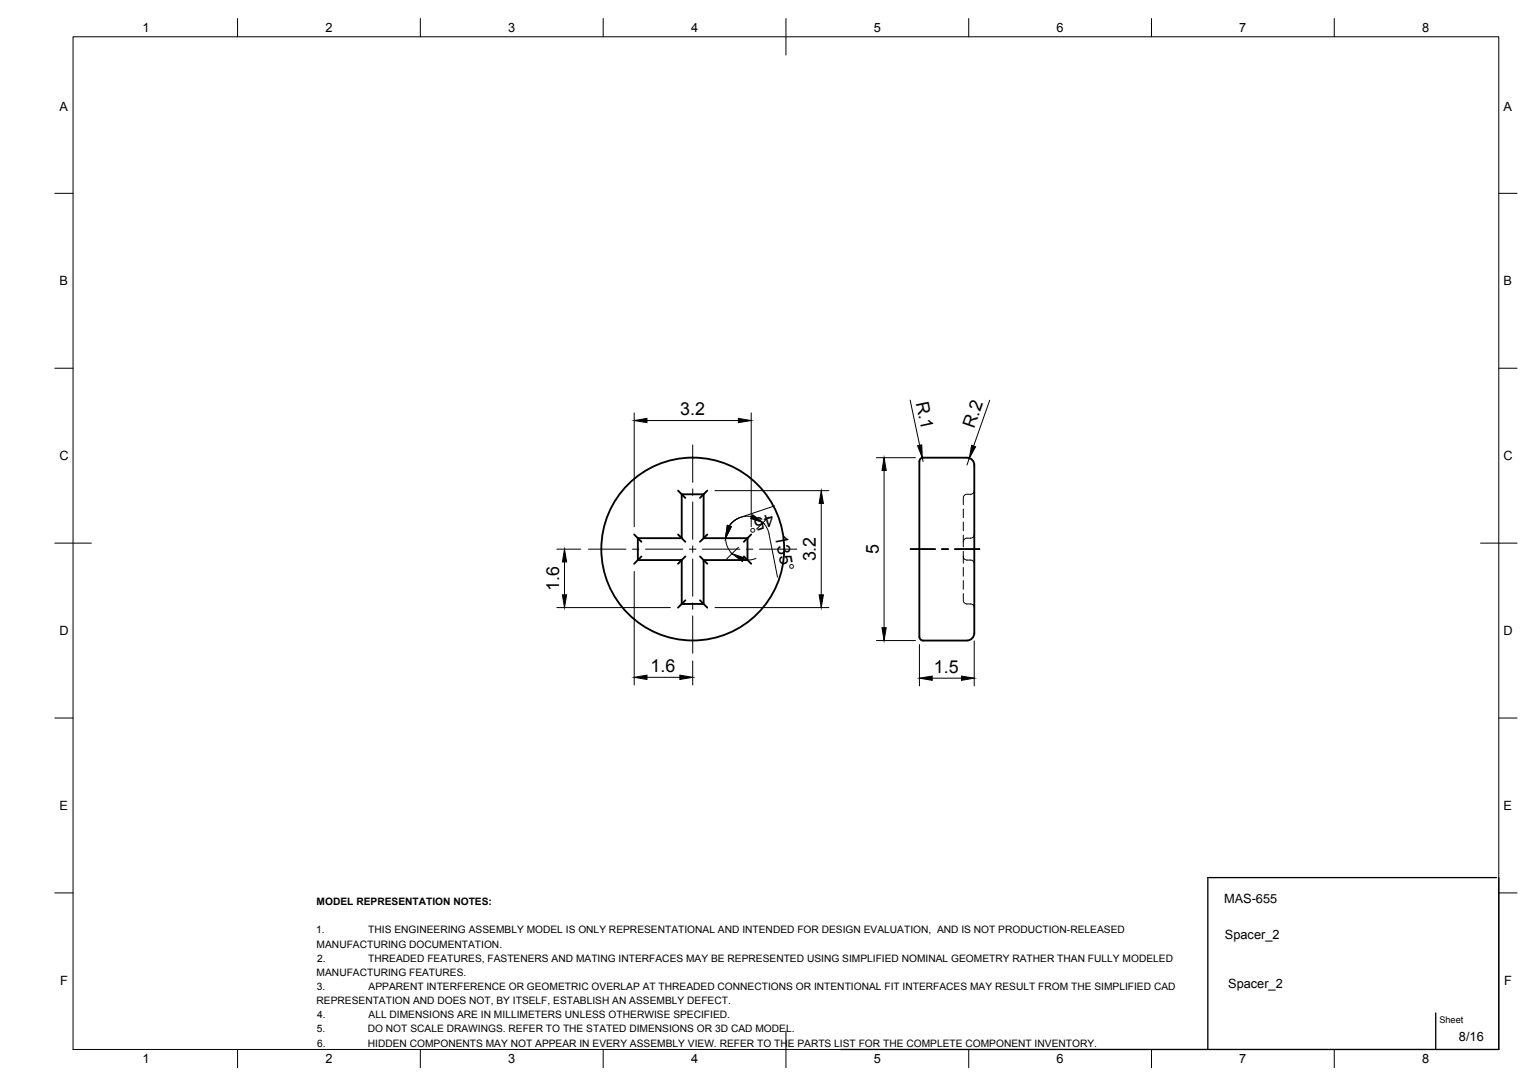
ISO-10303-21;
HEADER;
FILE_DESCRIPTION((''),'2;1');
FILE_NAME('Spacer_2.step','2026-10-09T11:34:15-07:00',(''),(''),'','','');
FILE_SCHEMA (('AUTOMOTIVE_DESIGN { 1 0 10303 214 3 1 1 }'));
ENDSEC;
DATA;
#10=MECHANICAL_DESIGN_GEOMETRIC_PRESENTATION_REPRESENTATION('',(#640),#117170);
#341=ELLIPSE('',#52296,0.141421356237297,0.1) ;
#342=ELLIPSE('',#52297,0.141421356237322,0.1) ;
#343=ELLIPSE('',#52299,0.141421356237322,0.1) ;
#344=ELLIPSE('',#52301,0.141421356237297,0.1) ;
#345=ELLIPSE('',#52303,0.141421356237322,0.1) ;
#346=ELLIPSE('',#52305,0.141421356237297,0.1) ;
#347=ELLIPSE('',#52307,0.141421356237322,0.1) ;
#348=ELLIPSE('',#52309,0.141421356237297,0.1) ;
#349=ELLIPSE('',#52311,0.141421356237322,0.1) ;
#350=ELLIPSE('',#52313,0.141421356237297,0.1) ;
#351=ELLIPSE('',#52315,0.141421356237322,0.1) ;
#352=ELLIPSE('',#52317,0.141421356237297,0.1) ;
#353=ELLIPSE('',#52336,0.141421356237297,0.1) ;
#354=ELLIPSE('',#52337,0.141421356237322,0.1) ;
#355=ELLIPSE('',#52339,0.141421356237322,0.1) ;
#356=ELLIPSE('',#52341,0.141421356237297,0.1) ;
#357=ELLIPSE('',#52343,0.141421356237322,0.1) ;
#358=ELLIPSE('',#52345,0.141421356237297,0.1) ;
#359=ELLIPSE('',#52347,0.141421356237297,0.1) ;
#360=ELLIPSE('',#52348,0.141421356237297,0.1) ;
#361=ELLIPSE('',#52350,0.141421356237322,0.1) ;
#362=ELLIPSE('',#52353,0.141421356237297,0.1) ;
#363=ELLIPSE('',#52355,0.141421356237322,0.1) ;
#364=ELLIPSE('',#52357,0.141421356237297,0.1) ;
#598=SHAPE_REPRESENTATION_RELATIONSHIP('SRR','None',#117253,#619) ;
#619=ADVANCED_BREP_SHAPE_REPRESENTATION('',(#661),#117161) ;
#640=STYLED_ITEM('',(#117355),#661) ;
#661=MANIFOLD_SOLID_BREP('Body1',#49069) ;
#735=FACE_BOUND('',#15452,.T.) ;
#2522=PLANE('',#52319) ;
#2523=PLANE('',#52320) ;
#2524=PLANE('',#52321) ;
#2525=PLANE('',#52322) ;
#2526=PLANE('',#52323) ;
#2527=PLANE('',#52324) ;
#2528=PLANE('',#52325) ;
#2529=PLANE('',#52334) ;
#2530=PLANE('',#52359) ;
#2531=PLANE('',#52360) ;
#2532=PLANE('',#52361) ;
#2533=PLANE('',#52362) ;
#2534=PLANE('',#52366) ;
#2535=PLANE('',#52367) ;
#2536=PLANE('',#52368) ;
#4427=LINE('',#88396,#7641) ;
#4428=LINE('',#88400,#7642) ;
#4429=LINE('',#88404,#7643) ;
#4430=LINE('',#88407,#7644) ;
#4431=LINE('',#88410,#7645) ;
#4432=LINE('',#88413,#7646) ;
#4433=LINE('',#88416,#7647) ;
#4434=LINE('',#88419,#7648) ;
#4435=LINE('',#88422,#7649) ;
#4436=LINE('',#88425,#7650) ;
#4437=LINE('',#88428,#7651) ;
#4438=LINE('',#88430,#7652) ;
#4439=LINE('',#88434,#7653) ;
#4440=LINE('',#88436,#7654) ;
#4441=LINE('',#88440,#7655) ;
#4442=LINE('',#88442,#7656) ;
#4443=LINE('',#88446,#7657) ;
#4444=LINE('',#88448,#7658) ;
#4445=LINE('',#88452,#7659) ;
#4446=LINE('',#88454,#7660) ;
#4447=LINE('',#88458,#7661) ;
#4448=LINE('',#88460,#7662) ;
#4449=LINE('',#88463,#7663) ;
#4450=LINE('',#88464,#7664) ;
#4451=LINE('',#88467,#7665) ;
#4452=LINE('',#88469,#7666) ;
#4453=LINE('',#88470,#7667) ;
#4454=LINE('',#88473,#7668) ;
#4455=LINE('',#88474,#7669) ;
#4456=LINE('',#88477,#7670) ;
#4457=LINE('',#88478,#7671) ;
#4458=LINE('',#88481,#7672) ;
#4459=LINE('',#88482,#7673) ;
#4460=LINE('',#88485,#7674) ;
#4461=LINE('',#88486,#7675) ;
#4462=LINE('',#88489,#7676) ;
#4463=LINE('',#88490,#7677) ;
#4464=LINE('',#88502,#7678) ;
#4465=LINE('',#88510,#7679) ;
#4466=LINE('',#88515,#7680) ;
#4467=LINE('',#88519,#7681) ;
#4468=LINE('',#88523,#7682) ;
#4469=LINE('',#88527,#7683) ;
#4470=LINE('',#88530,#7684) ;
#4471=LINE('',#88534,#7685) ;
#4472=LINE('',#88538,#7686) ;
#4473=LINE('',#88542,#7687) ;
#4474=LINE('',#88544,#7688) ;
#4475=LINE('',#88547,#7689) ;
#4476=LINE('',#88548,#7690) ;
#4477=LINE('',#88551,#7691) ;
#4478=LINE('',#88553,#7692) ;
#4479=LINE('',#88556,#7693) ;
#4480=LINE('',#88558,#7694) ;
#4481=LINE('',#88562,#7695) ;
#4482=LINE('',#88565,#7696) ;
#4483=LINE('',#88567,#7697) ;
#4484=LINE('',#88569,#7698) ;
#4485=LINE('',#88571,#7699) ;
#4486=LINE('',#88578,#7700) ;
#4487=LINE('',#88580,#7701) ;
#7641=VECTOR('',#62464,10.) ;
#7642=VECTOR('',#62467,10.) ;
#7643=VECTOR('',#62472,10.) ;
#7644=VECTOR('',#62475,10.) ;
#7645=VECTOR('',#62478,10.) ;
#7646=VECTOR('',#62481,10.) ;
#7647=VECTOR('',#62484,10.) ;
#7648=VECTOR('',#62487,10.) ;
#7649=VECTOR('',#62490,10.) ;
#7650=VECTOR('',#62493,10.) ;
#7651=VECTOR('',#62496,10.) ;
#7652=VECTOR('',#62497,10.) ;
#7653=VECTOR('',#62502,10.) ;
#7654=VECTOR('',#62503,10.) ;
#7655=VECTOR('',#62508,10.) ;
#7656=VECTOR('',#62509,10.) ;
#7657=VECTOR('',#62514,10.) ;
#7658=VECTOR('',#62515,10.) ;
#7659=VECTOR('',#62520,10.) ;
#7660=VECTOR('',#62521,10.) ;
#7661=VECTOR('',#62526,10.) ;
#7662=VECTOR('',#62527,10.) ;
#7663=VECTOR('',#62532,10.) ;
#7664=VECTOR('',#62533,10.) ;
#7665=VECTOR('',#62536,10.) ;
#7666=VECTOR('',#62537,10.) ;
#7667=VECTOR('',#62538,10.) ;
#7668=VECTOR('',#62541,10.) ;
#7669=VECTOR('',#62542,10.) ;
#7670=VECTOR('',#62545,10.) ;
#7671=VECTOR('',#62546,10.) ;
#7672=VECTOR('',#62549,10.) ;
#7673=VECTOR('',#62550,10.) ;
#7674=VECTOR('',#62553,10.) ;
#7675=VECTOR('',#62554,10.) ;
#7676=VECTOR('',#62557,10.) ;
#7677=VECTOR('',#62558,10.) ;
#7678=VECTOR('',#62573,2.49999999999999) ;
#7679=VECTOR('',#62582,10.) ;
#7680=VECTOR('',#62589,10.) ;
#7681=VECTOR('',#62594,10.) ;
#7682=VECTOR('',#62599,10.) ;
#7683=VECTOR('',#62604,10.) ;
#7684=VECTOR('',#62607,10.) ;
#7685=VECTOR('',#62610,10.) ;
#7686=VECTOR('',#62613,10.) ;
#7687=VECTOR('',#62618,10.) ;
#7688=VECTOR('',#62619,10.) ;
#7689=VECTOR('',#62624,10.) ;
#7690=VECTOR('',#62625,10.) ;
#7691=VECTOR('',#62628,10.) ;
#7692=VECTOR('',#62629,10.) ;
#7693=VECTOR('',#62634,10.) ;
#7694=VECTOR('',#62635,10.) ;
#7695=VECTOR('',#62640,10.) ;
#7696=VECTOR('',#62645,10.) ;
#7697=VECTOR('',#62648,10.) ;
#7698=VECTOR('',#62651,10.) ;
#7699=VECTOR('',#62654,10.) ;
#7700=VECTOR('',#62665,10.) ;
#7701=VECTOR('',#62668,10.) ;
#10065=CYLINDRICAL_SURFACE('',#52295,0.1) ;
#10066=CYLINDRICAL_SURFACE('',#52298,0.1) ;
#10067=CYLINDRICAL_SURFACE('',#52300,0.1) ;
#10068=CYLINDRICAL_SURFACE('',#52302,0.1) ;
#10069=CYLINDRICAL_SURFACE('',#52304,0.1) ;
#10070=CYLINDRICAL_SURFACE('',#52306,0.1) ;
#10071=CYLINDRICAL_SURFACE('',#52308,0.1) ;
#10072=CYLINDRICAL_SURFACE('',#52310,0.1) ;
#10073=CYLINDRICAL_SURFACE('',#52312,0.1) ;
#10074=CYLINDRICAL_SURFACE('',#52314,0.1) ;
#10075=CYLINDRICAL_SURFACE('',#52316,0.1) ;
#10076=CYLINDRICAL_SURFACE('',#52318,0.1) ;
#10077=CYLINDRICAL_SURFACE('',#52331,2.49999999999999) ;
#10078=CYLINDRICAL_SURFACE('',#52335,0.1) ;
#10079=CYLINDRICAL_SURFACE('',#52338,0.1) ;
#10080=CYLINDRICAL_SURFACE('',#52340,0.1) ;
#10081=CYLINDRICAL_SURFACE('',#52342,0.1) ;
#10082=CYLINDRICAL_SURFACE('',#52344,0.1) ;
#10083=CYLINDRICAL_SURFACE('',#52346,0.1) ;
#10084=CYLINDRICAL_SURFACE('',#52349,0.1) ;
#10085=CYLINDRICAL_SURFACE('',#52351,0.1) ;
#10086=CYLINDRICAL_SURFACE('',#52352,0.1) ;
#10087=CYLINDRICAL_SURFACE('',#52354,0.1) ;
#10088=CYLINDRICAL_SURFACE('',#52356,0.1) ;
#10089=CYLINDRICAL_SURFACE('',#52358,0.1) ;
#12257=FACE_OUTER_BOUND('',#15414,.T.) ;
#12258=FACE_OUTER_BOUND('',#15415,.T.) ;
#12259=FACE_OUTER_BOUND('',#15416,.T.) ;
#12260=FACE_OUTER_BOUND('',#15417,.T.) ;
#12261=FACE_OUTER_BOUND('',#15418,.T.) ;
#12262=FACE_OUTER_BOUND('',#15419,.T.) ;
#12263=FACE_OUTER_BOUND('',#15420,.T.) ;
#12264=FACE_OUTER_BOUND('',#15421,.T.) ;
#12265=FACE_OUTER_BOUND('',#15422,.T.) ;
#12266=FACE_OUTER_BOUND('',#15423,.T.) ;
#12267=FACE_OUTER_BOUND('',#15424,.T.) ;
#12268=FACE_OUTER_BOUND('',#15425,.T.) ;
#12269=FACE_OUTER_BOUND('',#15426,.T.) ;
#12270=FACE_OUTER_BOUND('',#15427,.T.) ;
#12271=FACE_OUTER_BOUND('',#15428,.T.) ;
#12272=FACE_OUTER_BOUND('',#15429,.T.) ;
#12273=FACE_OUTER_BOUND('',#15430,.T.) ;
#12274=FACE_OUTER_BOUND('',#15431,.T.) ;
#12275=FACE_OUTER_BOUND('',#15432,.T.) ;
#12276=FACE_OUTER_BOUND('',#15433,.T.) ;
#12277=FACE_OUTER_BOUND('',#15434,.T.) ;
#12278=FACE_OUTER_BOUND('',#15435,.T.) ;
#12279=FACE_OUTER_BOUND('',#15436,.T.) ;
#12280=FACE_OUTER_BOUND('',#15437,.T.) ;
#12281=FACE_OUTER_BOUND('',#15438,.T.) ;
#12282=FACE_OUTER_BOUND('',#15439,.T.) ;
#12283=FACE_OUTER_BOUND('',#15440,.T.) ;
#12284=FACE_OUTER_BOUND('',#15441,.T.) ;
#12285=FACE_OUTER_BOUND('',#15442,.T.) ;
#12286=FACE_OUTER_BOUND('',#15443,.T.) ;
#12287=FACE_OUTER_BOUND('',#15444,.T.) ;
#12288=FACE_OUTER_BOUND('',#15445,.T.) ;
#12289=FACE_OUTER_BOUND('',#15446,.T.) ;
#12290=FACE_OUTER_BOUND('',#15447,.T.) ;
#12291=FACE_OUTER_BOUND('',#15448,.T.) ;
#12292=FACE_OUTER_BOUND('',#15449,.T.) ;
#12293=FACE_OUTER_BOUND('',#15450,.T.) ;
#12294=FACE_OUTER_BOUND('',#15451,.T.) ;
#12295=FACE_OUTER_BOUND('',#15453,.T.) ;
#12296=FACE_OUTER_BOUND('',#15454,.T.) ;
#12297=FACE_OUTER_BOUND('',#15455,.T.) ;
#12298=FACE_OUTER_BOUND('',#15456,.T.) ;
#15414=EDGE_LOOP('',(#37928,#37929,#37930,#37931)) ;
#15415=EDGE_LOOP('',(#37932,#37933,#37934,#37935)) ;
#15416=EDGE_LOOP('',(#37936,#37937,#37938,#37939)) ;
#15417=EDGE_LOOP('',(#37940,#37941,#37942,#37943)) ;
#15418=EDGE_LOOP('',(#37944,#37945,#37946,#37947)) ;
#15419=EDGE_LOOP('',(#37948,#37949,#37950,#37951)) ;
#15420=EDGE_LOOP('',(#37952,#37953,#37954,#37955)) ;
#15421=EDGE_LOOP('',(#37956,#37957,#37958,#37959)) ;
#15422=EDGE_LOOP('',(#37960,#37961,#37962,#37963)) ;
#15423=EDGE_LOOP('',(#37964,#37965,#37966,#37967)) ;
#15424=EDGE_LOOP('',(#37968,#37969,#37970,#37971)) ;
#15425=EDGE_LOOP('',(#37972,#37973,#37974,#37975)) ;
#15426=EDGE_LOOP('',(#37976,#37977,#37978,#37979)) ;
#15427=EDGE_LOOP('',(#37980,#37981,#37982,#37983)) ;
#15428=EDGE_LOOP('',(#37984,#37985,#37986,#37987)) ;
#15429=EDGE_LOOP('',(#37988,#37989,#37990,#37991)) ;
#15430=EDGE_LOOP('',(#37992,#37993,#37994,#37995)) ;
#15431=EDGE_LOOP('',(#37996,#37997,#37998,#37999)) ;
#15432=EDGE_LOOP('',(#38000,#38001,#38002,#38003,#38004,#38005,#38006,#38007,
#38008,#38009,#38010,#38011)) ;
#15433=EDGE_LOOP('',(#38012,#38013,#38014,#38015,#38016)) ;
#15434=EDGE_LOOP('',(#38017,#38018,#38019,#38020,#38021,#38022)) ;
#15435=EDGE_LOOP('',(#38023)) ;
#15436=EDGE_LOOP('',(#38024,#38025,#38026,#38027)) ;
#15437=EDGE_LOOP('',(#38028,#38029,#38030,#38031)) ;
#15438=EDGE_LOOP('',(#38032,#38033,#38034,#38035)) ;
#15439=EDGE_LOOP('',(#38036,#38037,#38038,#38039)) ;
#15440=EDGE_LOOP('',(#38040,#38041,#38042,#38043)) ;
#15441=EDGE_LOOP('',(#38044,#38045,#38046,#38047)) ;
#15442=EDGE_LOOP('',(#38048,#38049,#38050,#38051)) ;
#15443=EDGE_LOOP('',(#38052,#38053,#38054,#38055)) ;
#15444=EDGE_LOOP('',(#38056,#38057,#38058,#38059)) ;
#15445=EDGE_LOOP('',(#38060,#38061,#38062,#38063)) ;
#15446=EDGE_LOOP('',(#38064,#38065,#38066,#38067)) ;
#15447=EDGE_LOOP('',(#38068,#38069,#38070,#38071)) ;
#15448=EDGE_LOOP('',(#38072,#38073,#38074,#38075)) ;
#15449=EDGE_LOOP('',(#38076,#38077,#38078,#38079)) ;
#15450=EDGE_LOOP('',(#38080,#38081,#38082,#38083)) ;
#15451=EDGE_LOOP('',(#38084)) ;
#15452=EDGE_LOOP('',(#38085,#38086,#38087,#38088,#38089,#38090,#38091,#38092,
#38093,#38094,#38095,#38096)) ;
#15453=EDGE_LOOP('',(#38097,#38098,#38099,#38100,#38101)) ;
#15454=EDGE_LOOP('',(#38102,#38103,#38104,#38105)) ;
#15455=EDGE_LOOP('',(#38106,#38107,#38108,#38109)) ;
#15456=EDGE_LOOP('',(#38110,#38111,#38112,#38113)) ;
#18493=CIRCLE('',#52327,2.39999999999999) ;
#18494=CIRCLE('',#52328,0.1) ;
#18495=CIRCLE('',#52329,2.49999999999999) ;
#18496=CIRCLE('',#52330,2.49999999999999) ;
#18497=CIRCLE('',#52332,2.49999999999999) ;
#18498=CIRCLE('',#52333,2.49999999999999) ;
#18499=CIRCLE('',#52363,2.29999999999999) ;
#18500=CIRCLE('',#52365,0.2) ;
#21561=VERTEX_POINT('',#88394) ;
#21562=VERTEX_POINT('',#88395) ;
#21563=VERTEX_POINT('',#88397) ;
#21564=VERTEX_POINT('',#88399) ;
#21565=VERTEX_POINT('',#88403) ;
#21566=VERTEX_POINT('',#88405) ;
#21567=VERTEX_POINT('',#88409) ;
#21568=VERTEX_POINT('',#88411) ;
#21569=VERTEX_POINT('',#88415) ;
#21570=VERTEX_POINT('',#88417) ;
#21571=VERTEX_POINT('',#88421) ;
#21572=VERTEX_POINT('',#88423) ;
#21573=VERTEX_POINT('',#88427) ;
#21574=VERTEX_POINT('',#88429) ;
#21575=VERTEX_POINT('',#88433) ;
#21576=VERTEX_POINT('',#88435) ;
#21577=VERTEX_POINT('',#88439) ;
#21578=VERTEX_POINT('',#88441) ;
#21579=VERTEX_POINT('',#88445) ;
#21580=VERTEX_POINT('',#88447) ;
#21581=VERTEX_POINT('',#88451) ;
#21582=VERTEX_POINT('',#88453) ;
#21583=VERTEX_POINT('',#88457) ;
#21584=VERTEX_POINT('',#88459) ;
#21585=VERTEX_POINT('',#88466) ;
#21586=VERTEX_POINT('',#88468) ;
#21587=VERTEX_POINT('',#88472) ;
#21588=VERTEX_POINT('',#88476) ;
#21589=VERTEX_POINT('',#88480) ;
#21590=VERTEX_POINT('',#88484) ;
#21591=VERTEX_POINT('',#88488) ;
#21592=VERTEX_POINT('',#88493) ;
#21593=VERTEX_POINT('',#88495) ;
#21594=VERTEX_POINT('',#88497) ;
#21595=VERTEX_POINT('',#88501) ;
#21596=VERTEX_POINT('',#88503) ;
#21597=VERTEX_POINT('',#88508) ;
#21598=VERTEX_POINT('',#88509) ;
#21599=VERTEX_POINT('',#88514) ;
#21600=VERTEX_POINT('',#88518) ;
#21601=VERTEX_POINT('',#88522) ;
#21602=VERTEX_POINT('',#88526) ;
#21603=VERTEX_POINT('',#88528) ;
#21604=VERTEX_POINT('',#88532) ;
#21605=VERTEX_POINT('',#88533) ;
#21606=VERTEX_POINT('',#88535) ;
#21607=VERTEX_POINT('',#88537) ;
#21608=VERTEX_POINT('',#88541) ;
#21609=VERTEX_POINT('',#88543) ;
#21610=VERTEX_POINT('',#88550) ;
#21611=VERTEX_POINT('',#88552) ;
#21612=VERTEX_POINT('',#88557) ;
#21613=VERTEX_POINT('',#88561) ;
#21614=VERTEX_POINT('',#88573) ;
#27242=EDGE_CURVE('',#21561,#21562,#4427,.T.) ;
#27243=EDGE_CURVE('',#21562,#21563,#341,.T.) ;
#27244=EDGE_CURVE('',#21563,#21564,#4428,.T.) ;
#27245=EDGE_CURVE('',#21561,#21564,#342,.T.) ;
#27246=EDGE_CURVE('',#21562,#21565,#4429,.T.) ;
#27247=EDGE_CURVE('',#21565,#21566,#343,.T.) ;
#27248=EDGE_CURVE('',#21566,#21563,#4430,.T.) ;
#27249=EDGE_CURVE('',#21565,#21567,#4431,.T.) ;
#27250=EDGE_CURVE('',#21567,#21568,#344,.T.) ;
#27251=EDGE_CURVE('',#21568,#21566,#4432,.T.) ;
#27252=EDGE_CURVE('',#21567,#21569,#4433,.T.) ;
#27253=EDGE_CURVE('',#21569,#21570,#345,.T.) ;
#27254=EDGE_CURVE('',#21570,#21568,#4434,.T.) ;
#27255=EDGE_CURVE('',#21569,#21571,#4435,.T.) ;
#27256=EDGE_CURVE('',#21571,#21572,#346,.T.) ;
#27257=EDGE_CURVE('',#21572,#21570,#4436,.T.) ;
#27258=EDGE_CURVE('',#21573,#21572,#4437,.T.) ;
#27259=EDGE_CURVE('',#21571,#21574,#4438,.T.) ;
#27260=EDGE_CURVE('',#21574,#21573,#347,.T.) ;
#27261=EDGE_CURVE('',#21575,#21573,#4439,.T.) ;
#27262=EDGE_CURVE('',#21574,#21576,#4440,.T.) ;
#27263=EDGE_CURVE('',#21576,#21575,#348,.T.) ;
#27264=EDGE_CURVE('',#21577,#21575,#4441,.T.) ;
#27265=EDGE_CURVE('',#21576,#21578,#4442,.T.) ;
#27266=EDGE_CURVE('',#21578,#21577,#349,.T.) ;
#27267=EDGE_CURVE('',#21579,#21577,#4443,.T.) ;
#27268=EDGE_CURVE('',#21578,#21580,#4444,.T.) ;
#27269=EDGE_CURVE('',#21580,#21579,#350,.T.) ;
#27270=EDGE_CURVE('',#21581,#21579,#4445,.T.) ;
#27271=EDGE_CURVE('',#21580,#21582,#4446,.T.) ;
#27272=EDGE_CURVE('',#21582,#21581,#351,.T.) ;
#27273=EDGE_CURVE('',#21583,#21581,#4447,.T.) ;
#27274=EDGE_CURVE('',#21582,#21584,#4448,.T.) ;
#27275=EDGE_CURVE('',#21584,#21583,#352,.T.) ;
#27276=EDGE_CURVE('',#21564,#21583,#4449,.T.) ;
#27277=EDGE_CURVE('',#21584,#21561,#4450,.T.) ;
#27278=EDGE_CURVE('',#21585,#21577,#4451,.T.) ;
#27279=EDGE_CURVE('',#21586,#21585,#4452,.T.) ;
#27280=EDGE_CURVE('',#21586,#21575,#4453,.T.) ;
#27281=EDGE_CURVE('',#21587,#21579,#4454,.T.) ;
#27282=EDGE_CURVE('',#21585,#21587,#4455,.T.) ;
#27283=EDGE_CURVE('',#21588,#21581,#4456,.T.) ;
#27284=EDGE_CURVE('',#21587,#21588,#4457,.T.) ;
#27285=EDGE_CURVE('',#21589,#21583,#4458,.T.) ;
#27286=EDGE_CURVE('',#21588,#21589,#4459,.T.) ;
#27287=EDGE_CURVE('',#21590,#21564,#4460,.T.) ;
#27288=EDGE_CURVE('',#21589,#21590,#4461,.T.) ;
#27289=EDGE_CURVE('',#21591,#21563,#4462,.T.) ;
#27290=EDGE_CURVE('',#21590,#21591,#4463,.T.) ;
#27291=EDGE_CURVE('',#21592,#21592,#18493,.T.) ;
#27292=EDGE_CURVE('',#21592,#21593,#18494,.T.) ;
#27293=EDGE_CURVE('',#21593,#21594,#18495,.T.) ;
#27294=EDGE_CURVE('',#21594,#21593,#18496,.T.) ;
#27295=EDGE_CURVE('',#21594,#21595,#4464,.T.) ;
#27296=EDGE_CURVE('',#21596,#21595,#18497,.T.) ;
#27297=EDGE_CURVE('',#21595,#21596,#18498,.T.) ;
#27298=EDGE_CURVE('',#21597,#21598,#4465,.T.) ;
#27299=EDGE_CURVE('',#21598,#21588,#353,.T.) ;
#27300=EDGE_CURVE('',#21597,#21589,#354,.T.) ;
#27301=EDGE_CURVE('',#21598,#21599,#4466,.T.) ;
#27302=EDGE_CURVE('',#21599,#21587,#355,.T.) ;
#27303=EDGE_CURVE('',#21599,#21600,#4467,.T.) ;
#27304=EDGE_CURVE('',#21600,#21585,#356,.T.) ;
#27305=EDGE_CURVE('',#21600,#21601,#4468,.T.) ;
#27306=EDGE_CURVE('',#21601,#21586,#357,.T.) ;
#27307=EDGE_CURVE('',#21601,#21602,#4469,.T.) ;
#27308=EDGE_CURVE('',#21602,#21603,#358,.T.) ;
#27309=EDGE_CURVE('',#21603,#21586,#4470,.T.) ;
#27310=EDGE_CURVE('',#21604,#21605,#4471,.T.) ;
#27311=EDGE_CURVE('',#21605,#21606,#359,.T.) ;
#27312=EDGE_CURVE('',#21606,#21607,#4472,.T.) ;
#27313=EDGE_CURVE('',#21607,#21604,#360,.T.) ;
#27314=EDGE_CURVE('',#21608,#21606,#4473,.T.) ;
#27315=EDGE_CURVE('',#21605,#21609,#4474,.T.) ;
#27316=EDGE_CURVE('',#21609,#21608,#361,.T.) ;
#27317=EDGE_CURVE('',#21602,#21604,#4475,.T.) ;
#27318=EDGE_CURVE('',#21607,#21603,#4476,.T.) ;
#27319=EDGE_CURVE('',#21610,#21608,#4477,.T.) ;
#27320=EDGE_CURVE('',#21609,#21611,#4478,.T.) ;
#27321=EDGE_CURVE('',#21611,#21610,#362,.T.) ;
#27322=EDGE_CURVE('',#21591,#21610,#4479,.T.) ;
#27323=EDGE_CURVE('',#21611,#21612,#4480,.T.) ;
#27324=EDGE_CURVE('',#21612,#21591,#363,.T.) ;
#27325=EDGE_CURVE('',#21612,#21613,#4481,.T.) ;
#27326=EDGE_CURVE('',#21613,#21590,#364,.T.) ;
#27327=EDGE_CURVE('',#21613,#21597,#4482,.T.) ;
#27328=EDGE_CURVE('',#21603,#21573,#4483,.T.) ;
#27329=EDGE_CURVE('',#21607,#21572,#4484,.T.) ;
#27330=EDGE_CURVE('',#21606,#21570,#4485,.T.) ;
#27331=EDGE_CURVE('',#21614,#21614,#18499,.T.) ;
#27332=EDGE_CURVE('',#21596,#21614,#18500,.T.) ;
#27333=EDGE_CURVE('',#21610,#21566,#4486,.T.) ;
#27334=EDGE_CURVE('',#21608,#21568,#4487,.T.) ;
#37928=ORIENTED_EDGE('',*,*,#27242,.T.) ;
#37929=ORIENTED_EDGE('',*,*,#27243,.T.) ;
#37930=ORIENTED_EDGE('',*,*,#27244,.T.) ;
#37931=ORIENTED_EDGE('',*,*,#27245,.F.) ;
#37932=ORIENTED_EDGE('',*,*,#27246,.T.) ;
#37933=ORIENTED_EDGE('',*,*,#27247,.T.) ;
#37934=ORIENTED_EDGE('',*,*,#27248,.T.) ;
#37935=ORIENTED_EDGE('',*,*,#27243,.F.) ;
#37936=ORIENTED_EDGE('',*,*,#27249,.T.) ;
#37937=ORIENTED_EDGE('',*,*,#27250,.T.) ;
#37938=ORIENTED_EDGE('',*,*,#27251,.T.) ;
#37939=ORIENTED_EDGE('',*,*,#27247,.F.) ;
#37940=ORIENTED_EDGE('',*,*,#27252,.T.) ;
#37941=ORIENTED_EDGE('',*,*,#27253,.T.) ;
#37942=ORIENTED_EDGE('',*,*,#27254,.T.) ;
#37943=ORIENTED_EDGE('',*,*,#27250,.F.) ;
#37944=ORIENTED_EDGE('',*,*,#27255,.T.) ;
#37945=ORIENTED_EDGE('',*,*,#27256,.T.) ;
#37946=ORIENTED_EDGE('',*,*,#27257,.T.) ;
#37947=ORIENTED_EDGE('',*,*,#27253,.F.) ;
#37948=ORIENTED_EDGE('',*,*,#27258,.T.) ;
#37949=ORIENTED_EDGE('',*,*,#27256,.F.) ;
#37950=ORIENTED_EDGE('',*,*,#27259,.T.) ;
#37951=ORIENTED_EDGE('',*,*,#27260,.T.) ;
#37952=ORIENTED_EDGE('',*,*,#27261,.T.) ;
#37953=ORIENTED_EDGE('',*,*,#27260,.F.) ;
#37954=ORIENTED_EDGE('',*,*,#27262,.T.) ;
#37955=ORIENTED_EDGE('',*,*,#27263,.T.) ;
#37956=ORIENTED_EDGE('',*,*,#27264,.T.) ;
#37957=ORIENTED_EDGE('',*,*,#27263,.F.) ;
#37958=ORIENTED_EDGE('',*,*,#27265,.T.) ;
#37959=ORIENTED_EDGE('',*,*,#27266,.T.) ;
#37960=ORIENTED_EDGE('',*,*,#27267,.T.) ;
#37961=ORIENTED_EDGE('',*,*,#27266,.F.) ;
#37962=ORIENTED_EDGE('',*,*,#27268,.T.) ;
#37963=ORIENTED_EDGE('',*,*,#27269,.T.) ;
#37964=ORIENTED_EDGE('',*,*,#27270,.T.) ;
#37965=ORIENTED_EDGE('',*,*,#27269,.F.) ;
#37966=ORIENTED_EDGE('',*,*,#27271,.T.) ;
#37967=ORIENTED_EDGE('',*,*,#27272,.T.) ;
#37968=ORIENTED_EDGE('',*,*,#27273,.T.) ;
#37969=ORIENTED_EDGE('',*,*,#27272,.F.) ;
#37970=ORIENTED_EDGE('',*,*,#27274,.T.) ;
#37971=ORIENTED_EDGE('',*,*,#27275,.T.) ;
#37972=ORIENTED_EDGE('',*,*,#27276,.T.) ;
#37973=ORIENTED_EDGE('',*,*,#27275,.F.) ;
#37974=ORIENTED_EDGE('',*,*,#27277,.T.) ;
#37975=ORIENTED_EDGE('',*,*,#27245,.T.) ;
#37976=ORIENTED_EDGE('',*,*,#27264,.F.) ;
#37977=ORIENTED_EDGE('',*,*,#27278,.F.) ;
#37978=ORIENTED_EDGE('',*,*,#27279,.F.) ;
#37979=ORIENTED_EDGE('',*,*,#27280,.T.) ;
#37980=ORIENTED_EDGE('',*,*,#27267,.F.) ;
#37981=ORIENTED_EDGE('',*,*,#27281,.F.) ;
#37982=ORIENTED_EDGE('',*,*,#27282,.F.) ;
#37983=ORIENTED_EDGE('',*,*,#27278,.T.) ;
#37984=ORIENTED_EDGE('',*,*,#27270,.F.) ;
#37985=ORIENTED_EDGE('',*,*,#27283,.F.) ;
#37986=ORIENTED_EDGE('',*,*,#27284,.F.) ;
#37987=ORIENTED_EDGE('',*,*,#27281,.T.) ;
#37988=ORIENTED_EDGE('',*,*,#27273,.F.) ;
#37989=ORIENTED_EDGE('',*,*,#27285,.F.) ;
#37990=ORIENTED_EDGE('',*,*,#27286,.F.) ;
#37991=ORIENTED_EDGE('',*,*,#27283,.T.) ;
#37992=ORIENTED_EDGE('',*,*,#27276,.F.) ;
#37993=ORIENTED_EDGE('',*,*,#27287,.F.) ;
#37994=ORIENTED_EDGE('',*,*,#27288,.F.) ;
#37995=ORIENTED_EDGE('',*,*,#27285,.T.) ;
#37996=ORIENTED_EDGE('',*,*,#27244,.F.) ;
#37997=ORIENTED_EDGE('',*,*,#27289,.F.) ;
#37998=ORIENTED_EDGE('',*,*,#27290,.F.) ;
#37999=ORIENTED_EDGE('',*,*,#27287,.T.) ;
#38000=ORIENTED_EDGE('',*,*,#27242,.F.) ;
#38001=ORIENTED_EDGE('',*,*,#27277,.F.) ;
#38002=ORIENTED_EDGE('',*,*,#27274,.F.) ;
#38003=ORIENTED_EDGE('',*,*,#27271,.F.) ;
#38004=ORIENTED_EDGE('',*,*,#27268,.F.) ;
#38005=ORIENTED_EDGE('',*,*,#27265,.F.) ;
#38006=ORIENTED_EDGE('',*,*,#27262,.F.) ;
#38007=ORIENTED_EDGE('',*,*,#27259,.F.) ;
#38008=ORIENTED_EDGE('',*,*,#27255,.F.) ;
#38009=ORIENTED_EDGE('',*,*,#27252,.F.) ;
#38010=ORIENTED_EDGE('',*,*,#27249,.F.) ;
#38011=ORIENTED_EDGE('',*,*,#27246,.F.) ;
#38012=ORIENTED_EDGE('',*,*,#27291,.T.) ;
#38013=ORIENTED_EDGE('',*,*,#27292,.T.) ;
#38014=ORIENTED_EDGE('',*,*,#27293,.T.) ;
#38015=ORIENTED_EDGE('',*,*,#27294,.T.) ;
#38016=ORIENTED_EDGE('',*,*,#27292,.F.) ;
#38017=ORIENTED_EDGE('',*,*,#27294,.F.) ;
#38018=ORIENTED_EDGE('',*,*,#27295,.T.) ;
#38019=ORIENTED_EDGE('',*,*,#27296,.F.) ;
#38020=ORIENTED_EDGE('',*,*,#27297,.F.) ;
#38021=ORIENTED_EDGE('',*,*,#27295,.F.) ;
#38022=ORIENTED_EDGE('',*,*,#27293,.F.) ;
#38023=ORIENTED_EDGE('',*,*,#27291,.F.) ;
#38024=ORIENTED_EDGE('',*,*,#27298,.T.) ;
#38025=ORIENTED_EDGE('',*,*,#27299,.T.) ;
#38026=ORIENTED_EDGE('',*,*,#27286,.T.) ;
#38027=ORIENTED_EDGE('',*,*,#27300,.F.) ;
#38028=ORIENTED_EDGE('',*,*,#27301,.T.) ;
#38029=ORIENTED_EDGE('',*,*,#27302,.T.) ;
#38030=ORIENTED_EDGE('',*,*,#27284,.T.) ;
#38031=ORIENTED_EDGE('',*,*,#27299,.F.) ;
#38032=ORIENTED_EDGE('',*,*,#27303,.T.) ;
#38033=ORIENTED_EDGE('',*,*,#27304,.T.) ;
#38034=ORIENTED_EDGE('',*,*,#27282,.T.) ;
#38035=ORIENTED_EDGE('',*,*,#27302,.F.) ;
#38036=ORIENTED_EDGE('',*,*,#27305,.T.) ;
#38037=ORIENTED_EDGE('',*,*,#27306,.T.) ;
#38038=ORIENTED_EDGE('',*,*,#27279,.T.) ;
#38039=ORIENTED_EDGE('',*,*,#27304,.F.) ;
#38040=ORIENTED_EDGE('',*,*,#27307,.T.) ;
#38041=ORIENTED_EDGE('',*,*,#27308,.T.) ;
#38042=ORIENTED_EDGE('',*,*,#27309,.T.) ;
#38043=ORIENTED_EDGE('',*,*,#27306,.F.) ;
#38044=ORIENTED_EDGE('',*,*,#27310,.T.) ;
#38045=ORIENTED_EDGE('',*,*,#27311,.T.) ;
#38046=ORIENTED_EDGE('',*,*,#27312,.T.) ;
#38047=ORIENTED_EDGE('',*,*,#27313,.T.) ;
#38048=ORIENTED_EDGE('',*,*,#27314,.T.) ;
#38049=ORIENTED_EDGE('',*,*,#27311,.F.) ;
#38050=ORIENTED_EDGE('',*,*,#27315,.T.) ;
#38051=ORIENTED_EDGE('',*,*,#27316,.T.) ;
#38052=ORIENTED_EDGE('',*,*,#27317,.T.) ;
#38053=ORIENTED_EDGE('',*,*,#27313,.F.) ;
#38054=ORIENTED_EDGE('',*,*,#27318,.T.) ;
#38055=ORIENTED_EDGE('',*,*,#27308,.F.) ;
#38056=ORIENTED_EDGE('',*,*,#27319,.T.) ;
#38057=ORIENTED_EDGE('',*,*,#27316,.F.) ;
#38058=ORIENTED_EDGE('',*,*,#27320,.T.) ;
#38059=ORIENTED_EDGE('',*,*,#27321,.T.) ;
#38060=ORIENTED_EDGE('',*,*,#27322,.T.) ;
#38061=ORIENTED_EDGE('',*,*,#27321,.F.) ;
#38062=ORIENTED_EDGE('',*,*,#27323,.T.) ;
#38063=ORIENTED_EDGE('',*,*,#27324,.T.) ;
#38064=ORIENTED_EDGE('',*,*,#27290,.T.) ;
#38065=ORIENTED_EDGE('',*,*,#27324,.F.) ;
#38066=ORIENTED_EDGE('',*,*,#27325,.T.) ;
#38067=ORIENTED_EDGE('',*,*,#27326,.T.) ;
#38068=ORIENTED_EDGE('',*,*,#27288,.T.) ;
#38069=ORIENTED_EDGE('',*,*,#27326,.F.) ;
#38070=ORIENTED_EDGE('',*,*,#27327,.T.) ;
#38071=ORIENTED_EDGE('',*,*,#27300,.T.) ;
#38072=ORIENTED_EDGE('',*,*,#27261,.F.) ;
#38073=ORIENTED_EDGE('',*,*,#27280,.F.) ;
#38074=ORIENTED_EDGE('',*,*,#27309,.F.) ;
#38075=ORIENTED_EDGE('',*,*,#27328,.T.) ;
#38076=ORIENTED_EDGE('',*,*,#27258,.F.) ;
#38077=ORIENTED_EDGE('',*,*,#27328,.F.) ;
#38078=ORIENTED_EDGE('',*,*,#27318,.F.) ;
#38079=ORIENTED_EDGE('',*,*,#27329,.T.) ;
#38080=ORIENTED_EDGE('',*,*,#27257,.F.) ;
#38081=ORIENTED_EDGE('',*,*,#27329,.F.) ;
#38082=ORIENTED_EDGE('',*,*,#27312,.F.) ;
#38083=ORIENTED_EDGE('',*,*,#27330,.T.) ;
#38084=ORIENTED_EDGE('',*,*,#27331,.F.) ;
#38085=ORIENTED_EDGE('',*,*,#27310,.F.) ;
#38086=ORIENTED_EDGE('',*,*,#27317,.F.) ;
#38087=ORIENTED_EDGE('',*,*,#27307,.F.) ;
#38088=ORIENTED_EDGE('',*,*,#27305,.F.) ;
#38089=ORIENTED_EDGE('',*,*,#27303,.F.) ;
#38090=ORIENTED_EDGE('',*,*,#27301,.F.) ;
#38091=ORIENTED_EDGE('',*,*,#27298,.F.) ;
#38092=ORIENTED_EDGE('',*,*,#27327,.F.) ;
#38093=ORIENTED_EDGE('',*,*,#27325,.F.) ;
#38094=ORIENTED_EDGE('',*,*,#27323,.F.) ;
#38095=ORIENTED_EDGE('',*,*,#27320,.F.) ;
#38096=ORIENTED_EDGE('',*,*,#27315,.F.) ;
#38097=ORIENTED_EDGE('',*,*,#27296,.T.) ;
#38098=ORIENTED_EDGE('',*,*,#27297,.T.) ;
#38099=ORIENTED_EDGE('',*,*,#27332,.T.) ;
#38100=ORIENTED_EDGE('',*,*,#27331,.T.) ;
#38101=ORIENTED_EDGE('',*,*,#27332,.F.) ;
#38102=ORIENTED_EDGE('',*,*,#27248,.F.) ;
#38103=ORIENTED_EDGE('',*,*,#27333,.F.) ;
#38104=ORIENTED_EDGE('',*,*,#27322,.F.) ;
#38105=ORIENTED_EDGE('',*,*,#27289,.T.) ;
#38106=ORIENTED_EDGE('',*,*,#27251,.F.) ;
#38107=ORIENTED_EDGE('',*,*,#27334,.F.) ;
#38108=ORIENTED_EDGE('',*,*,#27319,.F.) ;
#38109=ORIENTED_EDGE('',*,*,#27333,.T.) ;
#38110=ORIENTED_EDGE('',*,*,#27254,.F.) ;
#38111=ORIENTED_EDGE('',*,*,#27330,.F.) ;
#38112=ORIENTED_EDGE('',*,*,#27314,.F.) ;
#38113=ORIENTED_EDGE('',*,*,#27334,.T.) ;
#45709=TOROIDAL_SURFACE('',#52326,2.39999999999999,0.1) ;
#45710=TOROIDAL_SURFACE('',#52364,2.29999999999999,0.2) ;
#47475=ADVANCED_FACE('',(#12257),#10065,.F.) ;
#47476=ADVANCED_FACE('',(#12258),#10066,.F.) ;
#47477=ADVANCED_FACE('',(#12259),#10067,.F.) ;
#47478=ADVANCED_FACE('',(#12260),#10068,.F.) ;
#47479=ADVANCED_FACE('',(#12261),#10069,.F.) ;
#47480=ADVANCED_FACE('',(#12262),#10070,.F.) ;
#47481=ADVANCED_FACE('',(#12263),#10071,.F.) ;
#47482=ADVANCED_FACE('',(#12264),#10072,.F.) ;
#47483=ADVANCED_FACE('',(#12265),#10073,.F.) ;
#47484=ADVANCED_FACE('',(#12266),#10074,.F.) ;
#47485=ADVANCED_FACE('',(#12267),#10075,.F.) ;
#47486=ADVANCED_FACE('',(#12268),#10076,.F.) ;
#47487=ADVANCED_FACE('',(#12269),#2522,.F.) ;
#47488=ADVANCED_FACE('',(#12270),#2523,.F.) ;
#47489=ADVANCED_FACE('',(#12271),#2524,.F.) ;
#47490=ADVANCED_FACE('',(#12272),#2525,.F.) ;
#47491=ADVANCED_FACE('',(#12273),#2526,.F.) ;
#47492=ADVANCED_FACE('',(#12274),#2527,.F.) ;
#47493=ADVANCED_FACE('',(#12275),#2528,.F.) ;
#47494=ADVANCED_FACE('',(#12276),#45709,.T.) ;
#47495=ADVANCED_FACE('',(#12277),#10077,.T.) ;
#47496=ADVANCED_FACE('',(#12278),#2529,.T.) ;
#47497=ADVANCED_FACE('',(#12279),#10078,.T.) ;
#47498=ADVANCED_FACE('',(#12280),#10079,.T.) ;
#47499=ADVANCED_FACE('',(#12281),#10080,.T.) ;
#47500=ADVANCED_FACE('',(#12282),#10081,.T.) ;
#47501=ADVANCED_FACE('',(#12283),#10082,.T.) ;
#47502=ADVANCED_FACE('',(#12284),#10083,.T.) ;
#47503=ADVANCED_FACE('',(#12285),#10084,.T.) ;
#47504=ADVANCED_FACE('',(#12286),#10085,.T.) ;
#47505=ADVANCED_FACE('',(#12287),#10086,.T.) ;
#47506=ADVANCED_FACE('',(#12288),#10087,.T.) ;
#47507=ADVANCED_FACE('',(#12289),#10088,.T.) ;
#47508=ADVANCED_FACE('',(#12290),#10089,.T.) ;
#47509=ADVANCED_FACE('',(#12291),#2530,.F.) ;
#47510=ADVANCED_FACE('',(#12292),#2531,.F.) ;
#47511=ADVANCED_FACE('',(#12293),#2532,.F.) ;
#47512=ADVANCED_FACE('',(#12294,#735),#2533,.F.) ;
#47513=ADVANCED_FACE('',(#12295),#45710,.T.) ;
#47514=ADVANCED_FACE('',(#12296),#2534,.F.) ;
#47515=ADVANCED_FACE('',(#12297),#2535,.F.) ;
#47516=ADVANCED_FACE('',(#12298),#2536,.F.) ;
#49069=CLOSED_SHELL('',(#47475,#47476,#47477,#47478,#47479,#47480,#47481,
#47482,#47483,#47484,#47485,#47486,#47487,#47488,#47489,#47490,#47491,#47492,
#47493,#47494,#47495,#47496,#47497,#47498,#47499,#47500,#47501,#47502,#47503,
#47504,#47505,#47506,#47507,#47508,#47509,#47510,#47511,#47512,#47513,#47514,
#47515,#47516)) ;
#52294=AXIS2_PLACEMENT_3D('',#88392,#62460,#62461) ;
#52295=AXIS2_PLACEMENT_3D('',#88393,#62462,#62463) ;
#52296=AXIS2_PLACEMENT_3D('',#88398,#62465,#62466) ;
#52297=AXIS2_PLACEMENT_3D('',#88401,#62468,#62469) ;
#52298=AXIS2_PLACEMENT_3D('',#88402,#62470,#62471) ;
#52299=AXIS2_PLACEMENT_3D('',#88406,#62473,#62474) ;
#52300=AXIS2_PLACEMENT_3D('',#88408,#62476,#62477) ;
#52301=AXIS2_PLACEMENT_3D('',#88412,#62479,#62480) ;
#52302=AXIS2_PLACEMENT_3D('',#88414,#62482,#62483) ;
#52303=AXIS2_PLACEMENT_3D('',#88418,#62485,#62486) ;
#52304=AXIS2_PLACEMENT_3D('',#88420,#62488,#62489) ;
#52305=AXIS2_PLACEMENT_3D('',#88424,#62491,#62492) ;
#52306=AXIS2_PLACEMENT_3D('',#88426,#62494,#62495) ;
#52307=AXIS2_PLACEMENT_3D('',#88431,#62498,#62499) ;
#52308=AXIS2_PLACEMENT_3D('',#88432,#62500,#62501) ;
#52309=AXIS2_PLACEMENT_3D('',#88437,#62504,#62505) ;
#52310=AXIS2_PLACEMENT_3D('',#88438,#62506,#62507) ;
#52311=AXIS2_PLACEMENT_3D('',#88443,#62510,#62511) ;
#52312=AXIS2_PLACEMENT_3D('',#88444,#62512,#62513) ;
#52313=AXIS2_PLACEMENT_3D('',#88449,#62516,#62517) ;
#52314=AXIS2_PLACEMENT_3D('',#88450,#62518,#62519) ;
#52315=AXIS2_PLACEMENT_3D('',#88455,#62522,#62523) ;
#52316=AXIS2_PLACEMENT_3D('',#88456,#62524,#62525) ;
#52317=AXIS2_PLACEMENT_3D('',#88461,#62528,#62529) ;
#52318=AXIS2_PLACEMENT_3D('',#88462,#62530,#62531) ;
#52319=AXIS2_PLACEMENT_3D('',#88465,#62534,#62535) ;
#52320=AXIS2_PLACEMENT_3D('',#88471,#62539,#62540) ;
#52321=AXIS2_PLACEMENT_3D('',#88475,#62543,#62544) ;
#52322=AXIS2_PLACEMENT_3D('',#88479,#62547,#62548) ;
#52323=AXIS2_PLACEMENT_3D('',#88483,#62551,#62552) ;
#52324=AXIS2_PLACEMENT_3D('',#88487,#62555,#62556) ;
#52325=AXIS2_PLACEMENT_3D('',#88491,#62559,#62560) ;
#52326=AXIS2_PLACEMENT_3D('',#88492,#62561,#62562) ;
#52327=AXIS2_PLACEMENT_3D('',#88494,#62563,#62564) ;
#52328=AXIS2_PLACEMENT_3D('',#88496,#62565,#62566) ;
#52329=AXIS2_PLACEMENT_3D('',#88498,#62567,#62568) ;
#52330=AXIS2_PLACEMENT_3D('',#88499,#62569,#62570) ;
#52331=AXIS2_PLACEMENT_3D('',#88500,#62571,#62572) ;
#52332=AXIS2_PLACEMENT_3D('',#88504,#62574,#62575) ;
#52333=AXIS2_PLACEMENT_3D('',#88505,#62576,#62577) ;
#52334=AXIS2_PLACEMENT_3D('',#88506,#62578,#62579) ;
#52335=AXIS2_PLACEMENT_3D('',#88507,#62580,#62581) ;
#52336=AXIS2_PLACEMENT_3D('',#88511,#62583,#62584) ;
#52337=AXIS2_PLACEMENT_3D('',#88512,#62585,#62586) ;
#52338=AXIS2_PLACEMENT_3D('',#88513,#62587,#62588) ;
#52339=AXIS2_PLACEMENT_3D('',#88516,#62590,#62591) ;
#52340=AXIS2_PLACEMENT_3D('',#88517,#62592,#62593) ;
#52341=AXIS2_PLACEMENT_3D('',#88520,#62595,#62596) ;
#52342=AXIS2_PLACEMENT_3D('',#88521,#62597,#62598) ;
#52343=AXIS2_PLACEMENT_3D('',#88524,#62600,#62601) ;
#52344=AXIS2_PLACEMENT_3D('',#88525,#62602,#62603) ;
#52345=AXIS2_PLACEMENT_3D('',#88529,#62605,#62606) ;
#52346=AXIS2_PLACEMENT_3D('',#88531,#62608,#62609) ;
#52347=AXIS2_PLACEMENT_3D('',#88536,#62611,#62612) ;
#52348=AXIS2_PLACEMENT_3D('',#88539,#62614,#62615) ;
#52349=AXIS2_PLACEMENT_3D('',#88540,#62616,#62617) ;
#52350=AXIS2_PLACEMENT_3D('',#88545,#62620,#62621) ;
#52351=AXIS2_PLACEMENT_3D('',#88546,#62622,#62623) ;
#52352=AXIS2_PLACEMENT_3D('',#88549,#62626,#62627) ;
#52353=AXIS2_PLACEMENT_3D('',#88554,#62630,#62631) ;
#52354=AXIS2_PLACEMENT_3D('',#88555,#62632,#62633) ;
#52355=AXIS2_PLACEMENT_3D('',#88559,#62636,#62637) ;
#52356=AXIS2_PLACEMENT_3D('',#88560,#62638,#62639) ;
#52357=AXIS2_PLACEMENT_3D('',#88563,#62641,#62642) ;
#52358=AXIS2_PLACEMENT_3D('',#88564,#62643,#62644) ;
#52359=AXIS2_PLACEMENT_3D('',#88566,#62646,#62647) ;
#52360=AXIS2_PLACEMENT_3D('',#88568,#62649,#62650) ;
#52361=AXIS2_PLACEMENT_3D('',#88570,#62652,#62653) ;
#52362=AXIS2_PLACEMENT_3D('',#88572,#62655,#62656) ;
#52363=AXIS2_PLACEMENT_3D('',#88574,#62657,#62658) ;
#52364=AXIS2_PLACEMENT_3D('',#88575,#62659,#62660) ;
#52365=AXIS2_PLACEMENT_3D('',#88576,#62661,#62662) ;
#52366=AXIS2_PLACEMENT_3D('',#88577,#62663,#62664) ;
#52367=AXIS2_PLACEMENT_3D('',#88579,#62666,#62667) ;
#52368=AXIS2_PLACEMENT_3D('',#88581,#62669,#62670) ;
#62460=DIRECTION('axis',(0.,0.,1.)) ;
#62461=DIRECTION('refdir',(1.,0.,0.)) ;
#62462=DIRECTION('center_axis',(-1.,0.,0.)) ;
#62463=DIRECTION('ref_axis',(0.,-0.707106781186485,-0.70710678118661)) ;
#62464=DIRECTION('',(-1.,0.,0.)) ;
#62465=DIRECTION('center_axis',(-0.70710678118661,0.707106781186485,0.)) ;
#62466=DIRECTION('ref_axis',(0.707106781186485,0.70710678118661,0.)) ;
#62467=DIRECTION('',(1.,0.,0.)) ;
#62468=DIRECTION('center_axis',(-0.70710678118661,0.707106781186485,0.)) ;
#62469=DIRECTION('ref_axis',(-0.707106781186485,-0.70710678118661,0.)) ;
#62470=DIRECTION('center_axis',(-1.41426179436738E-51,1.,0.)) ;
#62471=DIRECTION('ref_axis',(-0.707106781186548,-1.00003410517023E-51,-0.707106781186548)) ;
#62472=DIRECTION('',(-1.41426179436738E-51,1.,0.)) ;
#62473=DIRECTION('center_axis',(0.70710678118661,0.707106781186485,0.)) ;
#62474=DIRECTION('ref_axis',(0.707106781186485,-0.70710678118661,0.)) ;
#62475=DIRECTION('',(1.41426179436738E-51,-1.,0.)) ;
#62476=DIRECTION('center_axis',(1.,0.,0.)) ;
#62477=DIRECTION('ref_axis',(0.,0.707106781186485,-0.70710678118661)) ;
#62478=DIRECTION('',(1.,0.,0.)) ;
#62479=DIRECTION('center_axis',(0.70710678118661,0.707106781186485,0.)) ;
#62480=DIRECTION('ref_axis',(-0.707106781186485,0.70710678118661,0.)) ;
#62481=DIRECTION('',(-1.,0.,0.)) ;
#62482=DIRECTION('center_axis',(-1.41426179436738E-51,1.,0.)) ;
#62483=DIRECTION('ref_axis',(-0.707106781186548,-1.00003410517023E-51,-0.707106781186548)) ;
#62484=DIRECTION('',(-1.41426179436738E-51,1.,0.)) ;
#62485=DIRECTION('center_axis',(0.70710678118661,0.707106781186485,0.)) ;
#62486=DIRECTION('ref_axis',(0.707106781186485,-0.70710678118661,0.)) ;
#62487=DIRECTION('',(1.41426179436738E-51,-1.,0.)) ;
#62488=DIRECTION('center_axis',(1.,0.,0.)) ;
#62489=DIRECTION('ref_axis',(0.,0.707106781186485,-0.70710678118661)) ;
#62490=DIRECTION('',(1.,0.,0.)) ;
#62491=DIRECTION('center_axis',(0.70710678118661,-0.707106781186485,0.)) ;
#62492=DIRECTION('ref_axis',(-0.707106781186485,-0.70710678118661,0.)) ;
#62493=DIRECTION('',(-1.,0.,0.)) ;
#62494=DIRECTION('center_axis',(1.41426179436738E-51,-1.,0.)) ;
#62495=DIRECTION('ref_axis',(0.707106781186548,1.00003410517023E-51,-0.707106781186548)) ;
#62496=DIRECTION('',(-1.41426179436738E-51,1.,0.)) ;
#62497=DIRECTION('',(1.41426179436738E-51,-1.,0.)) ;
#62498=DIRECTION('center_axis',(0.70710678118661,-0.707106781186485,0.)) ;
#62499=DIRECTION('ref_axis',(0.707106781186485,0.70710678118661,0.)) ;
#62500=DIRECTION('center_axis',(1.,0.,0.)) ;
#62501=DIRECTION('ref_axis',(0.,0.707106781186485,-0.70710678118661)) ;
#62502=DIRECTION('',(-1.,0.,0.)) ;
#62503=DIRECTION('',(1.,0.,0.)) ;
#62504=DIRECTION('center_axis',(0.70710678118661,-0.707106781186485,0.)) ;
#62505=DIRECTION('ref_axis',(-0.707106781186485,-0.70710678118661,0.)) ;
#62506=DIRECTION('center_axis',(1.41426179436738E-51,-1.,0.)) ;
#62507=DIRECTION('ref_axis',(0.707106781186548,1.00003410517023E-51,-0.707106781186548)) ;
#62508=DIRECTION('',(-1.41426179436738E-51,1.,0.)) ;
#62509=DIRECTION('',(1.41426179436738E-51,-1.,0.)) ;
#62510=DIRECTION('center_axis',(-0.70710678118661,-0.707106781186485,0.)) ;
#62511=DIRECTION('ref_axis',(-0.707106781186485,0.70710678118661,0.)) ;
#62512=DIRECTION('center_axis',(-1.,0.,0.)) ;
#62513=DIRECTION('ref_axis',(0.,-0.707106781186485,-0.70710678118661)) ;
#62514=DIRECTION('',(1.,0.,0.)) ;
#62515=DIRECTION('',(-1.,0.,0.)) ;
#62516=DIRECTION('center_axis',(-0.70710678118661,-0.707106781186485,0.)) ;
#62517=DIRECTION('ref_axis',(0.707106781186485,-0.70710678118661,0.)) ;
#62518=DIRECTION('center_axis',(1.41426179436738E-51,-1.,0.)) ;
#62519=DIRECTION('ref_axis',(0.707106781186548,1.00003410517023E-51,-0.707106781186548)) ;
#62520=DIRECTION('',(-1.41426179436738E-51,1.,0.)) ;
#62521=DIRECTION('',(1.41426179436738E-51,-1.,0.)) ;
#62522=DIRECTION('center_axis',(-0.70710678118661,-0.707106781186485,0.)) ;
#62523=DIRECTION('ref_axis',(-0.707106781186485,0.70710678118661,0.)) ;
#62524=DIRECTION('center_axis',(-1.,0.,0.)) ;
#62525=DIRECTION('ref_axis',(0.,-0.707106781186485,-0.70710678118661)) ;
#62526=DIRECTION('',(1.,0.,0.)) ;
#62527=DIRECTION('',(-1.,0.,0.)) ;
#62528=DIRECTION('center_axis',(-0.70710678118661,0.707106781186485,0.)) ;
#62529=DIRECTION('ref_axis',(0.707106781186485,0.70710678118661,0.)) ;
#62530=DIRECTION('center_axis',(-1.41426179436738E-51,1.,0.)) ;
#62531=DIRECTION('ref_axis',(-0.707106781186548,-1.00003410517023E-51,-0.707106781186548)) ;
#62532=DIRECTION('',(1.41426179436738E-51,-1.,0.)) ;
#62533=DIRECTION('',(-1.41426179436738E-51,1.,0.)) ;
#62534=DIRECTION('center_axis',(1.,1.41426179436738E-51,0.)) ;
#62535=DIRECTION('ref_axis',(1.41426179436738E-51,-1.,-5.60383084497445E-34)) ;
#62536=DIRECTION('',(0.,0.,-1.)) ;
#62537=DIRECTION('',(1.41426179436738E-51,-1.,-5.60383084497445E-34)) ;
#62538=DIRECTION('',(0.,0.,-1.)) ;
#62539=DIRECTION('center_axis',(0.,-1.,0.)) ;
#62540=DIRECTION('ref_axis',(-1.,0.,-2.52374105052742E-18)) ;
#62541=DIRECTION('',(0.,0.,-1.)) ;
#62542=DIRECTION('',(-1.,0.,-2.52374105052742E-18)) ;
#62543=DIRECTION('center_axis',(1.,1.41426179436738E-51,0.)) ;
#62544=DIRECTION('ref_axis',(1.41426179436738E-51,-1.,-5.60383084497445E-34)) ;
#62545=DIRECTION('',(0.,0.,-1.)) ;
#62546=DIRECTION('',(1.41426179436738E-51,-1.,-5.60383084497445E-34)) ;
#62547=DIRECTION('center_axis',(0.,-1.,0.)) ;
#62548=DIRECTION('ref_axis',(-1.,0.,-2.52374105052742E-18)) ;
#62549=DIRECTION('',(0.,0.,-1.)) ;
#62550=DIRECTION('',(-1.,0.,-2.52374105052742E-18)) ;
#62551=DIRECTION('center_axis',(-1.,-1.41426179436738E-51,0.)) ;
#62552=DIRECTION('ref_axis',(-1.41426179436738E-51,1.,5.60383084497445E-34)) ;
#62553=DIRECTION('',(0.,0.,-1.)) ;
#62554=DIRECTION('',(-1.41426179436738E-51,1.,5.60383084497445E-34)) ;
#62555=DIRECTION('center_axis',(0.,-1.,0.)) ;
#62556=DIRECTION('ref_axis',(-1.,0.,-2.52374105052742E-18)) ;
#62557=DIRECTION('',(0.,0.,-1.)) ;
#62558=DIRECTION('',(-1.,0.,-2.52374105052742E-18)) ;
#62559=DIRECTION('center_axis',(0.,0.,-1.)) ;
#62560=DIRECTION('ref_axis',(-1.,0.,0.)) ;
#62561=DIRECTION('center_axis',(2.52374105052742E-18,5.60383084497445E-34,
-1.)) ;
#62562=DIRECTION('ref_axis',(-1.,0.,0.)) ;
#62563=DIRECTION('center_axis',(-2.52374105052742E-18,-5.60383084497445E-34,
1.)) ;
#62564=DIRECTION('ref_axis',(1.,-2.24153233798974E-35,2.52374105052742E-18)) ;
#62565=DIRECTION('center_axis',(0.,-1.,-5.60383084497445E-34)) ;
#62566=DIRECTION('ref_axis',(1.,0.,0.)) ;
#62567=DIRECTION('center_axis',(2.52374105052742E-18,5.60383084497445E-34,
-1.)) ;
#62568=DIRECTION('ref_axis',(1.,-2.24153233798974E-35,2.52374105052742E-18)) ;
#62569=DIRECTION('center_axis',(2.52374105052742E-18,5.60383084497445E-34,
-1.)) ;
#62570=DIRECTION('ref_axis',(1.,-2.24153233798974E-35,2.52374105052742E-18)) ;
#62571=DIRECTION('center_axis',(0.,0.,-1.)) ;
#62572=DIRECTION('ref_axis',(1.,0.,0.)) ;
#62573=DIRECTION('',(0.,0.,1.)) ;
#62574=DIRECTION('center_axis',(-2.52374105052742E-18,-5.60383084497445E-34,
1.)) ;
#62575=DIRECTION('ref_axis',(1.,4.48306467597958E-35,2.52374105052742E-18)) ;
#62576=DIRECTION('center_axis',(-2.52374105052742E-18,-5.60383084497445E-34,
1.)) ;
#62577=DIRECTION('ref_axis',(1.,4.48306467597958E-35,2.52374105052742E-18)) ;
#62578=DIRECTION('center_axis',(2.52374105052742E-18,5.60383084497445E-34,
-1.)) ;
#62579=DIRECTION('ref_axis',(1.,3.40207761657885E-68,2.52374105052742E-18)) ;
#62580=DIRECTION('center_axis',(-1.,0.,-2.52374105052742E-18)) ;
#62581=DIRECTION('ref_axis',(-1.78455441078696E-18,0.707106781186485,0.70710678118661)) ;
#62582=DIRECTION('',(1.,0.,2.52374105052742E-18)) ;
#62583=DIRECTION('center_axis',(-0.70710678118661,-0.707106781186485,0.)) ;
#62584=DIRECTION('ref_axis',(0.707106781186485,-0.70710678118661,3.56910882157392E-18)) ;
#62585=DIRECTION('center_axis',(-0.70710678118661,0.707106781186485,0.)) ;
#62586=DIRECTION('ref_axis',(-0.707106781186485,-0.70710678118661,-7.92501358220685E-34)) ;
#62587=DIRECTION('center_axis',(1.41426179436738E-51,-1.,-5.60383084497445E-34)) ;
#62588=DIRECTION('ref_axis',(-0.707106781186548,-3.96250679110377E-34,0.707106781186548)) ;
#62589=DIRECTION('',(-1.41426179436738E-51,1.,5.60383084497445E-34)) ;
#62590=DIRECTION('center_axis',(-0.70710678118661,-0.707106781186485,0.)) ;
#62591=DIRECTION('ref_axis',(-0.707106781186485,0.70710678118661,7.92501358220685E-34)) ;
#62592=DIRECTION('center_axis',(-1.,0.,-2.52374105052742E-18)) ;
#62593=DIRECTION('ref_axis',(-1.78455441078696E-18,0.707106781186485,0.70710678118661)) ;
#62594=DIRECTION('',(1.,0.,2.52374105052742E-18)) ;
#62595=DIRECTION('center_axis',(-0.70710678118661,-0.707106781186485,0.)) ;
#62596=DIRECTION('ref_axis',(0.707106781186485,-0.70710678118661,3.56910882157392E-18)) ;
#62597=DIRECTION('center_axis',(1.41426179436738E-51,-1.,-5.60383084497445E-34)) ;
#62598=DIRECTION('ref_axis',(-0.707106781186548,-3.96250679110377E-34,0.707106781186548)) ;
#62599=DIRECTION('',(-1.41426179436738E-51,1.,5.60383084497445E-34)) ;
#62600=DIRECTION('center_axis',(0.70710678118661,-0.707106781186485,0.)) ;
#62601=DIRECTION('ref_axis',(0.707106781186485,0.70710678118661,7.92501358220685E-34)) ;
#62602=DIRECTION('center_axis',(1.,0.,2.52374105052742E-18)) ;
#62603=DIRECTION('ref_axis',(-1.78455441078696E-18,-0.707106781186485,0.70710678118661)) ;
#62604=DIRECTION('',(-1.,0.,-2.52374105052742E-18)) ;
#62605=DIRECTION('center_axis',(0.70710678118661,-0.707106781186485,0.)) ;
#62606=DIRECTION('ref_axis',(-0.707106781186485,-0.70710678118661,-3.56910882157392E-18)) ;
#62607=DIRECTION('',(1.,0.,2.52374105052742E-18)) ;
#62608=DIRECTION('center_axis',(1.,0.,2.52374105052742E-18)) ;
#62609=DIRECTION('ref_axis',(-1.78455441078696E-18,-0.707106781186485,0.70710678118661)) ;
#62610=DIRECTION('',(-1.,0.,-2.52374105052742E-18)) ;
#62611=DIRECTION('center_axis',(0.70710678118661,0.707106781186485,0.)) ;
#62612=DIRECTION('ref_axis',(-0.707106781186485,0.70710678118661,-3.56910882157392E-18)) ;
#62613=DIRECTION('',(1.,0.,2.52374105052742E-18)) ;
#62614=DIRECTION('center_axis',(-0.70710678118661,0.707106781186485,0.)) ;
#62615=DIRECTION('ref_axis',(-0.707106781186485,-0.70710678118661,-3.56910882157392E-18)) ;
#62616=DIRECTION('center_axis',(-1.41426179436738E-51,1.,5.60383084497445E-34)) ;
#62617=DIRECTION('ref_axis',(0.707106781186548,-3.96250679110377E-34,0.707106781186548)) ;
#62618=DIRECTION('',(-1.41426179436738E-51,1.,5.60383084497445E-34)) ;
#62619=DIRECTION('',(1.41426179436738E-51,-1.,-5.60383084497445E-34)) ;
#62620=DIRECTION('center_axis',(0.70710678118661,0.707106781186485,0.)) ;
#62621=DIRECTION('ref_axis',(0.707106781186485,-0.70710678118661,-7.92501358220685E-34)) ;
#62622=DIRECTION('center_axis',(1.41426179436738E-51,-1.,-5.60383084497445E-34)) ;
#62623=DIRECTION('ref_axis',(-0.707106781186548,-3.96250679110377E-34,0.707106781186548)) ;
#62624=DIRECTION('',(-1.41426179436738E-51,1.,5.60383084497445E-34)) ;
#62625=DIRECTION('',(1.41426179436738E-51,-1.,-5.60383084497445E-34)) ;
#62626=DIRECTION('center_axis',(1.,0.,2.52374105052742E-18)) ;
#62627=DIRECTION('ref_axis',(-1.78455441078696E-18,-0.707106781186485,0.70710678118661)) ;
#62628=DIRECTION('',(1.,0.,2.52374105052742E-18)) ;
#62629=DIRECTION('',(-1.,0.,-2.52374105052742E-18)) ;
#62630=DIRECTION('center_axis',(0.70710678118661,0.707106781186485,0.)) ;
#62631=DIRECTION('ref_axis',(-0.707106781186485,0.70710678118661,-3.56910882157392E-18)) ;
#62632=DIRECTION('center_axis',(-1.41426179436738E-51,1.,5.60383084497445E-34)) ;
#62633=DIRECTION('ref_axis',(0.707106781186548,-3.96250679110377E-34,0.707106781186548)) ;
#62634=DIRECTION('',(-1.41426179436738E-51,1.,5.60383084497445E-34)) ;
#62635=DIRECTION('',(1.41426179436738E-51,-1.,-5.60383084497445E-34)) ;
#62636=DIRECTION('center_axis',(-0.70710678118661,0.707106781186485,0.)) ;
#62637=DIRECTION('ref_axis',(-0.707106781186485,-0.70710678118661,-7.92501358220685E-34)) ;
#62638=DIRECTION('center_axis',(-1.,0.,-2.52374105052742E-18)) ;
#62639=DIRECTION('ref_axis',(-1.78455441078696E-18,0.707106781186485,0.70710678118661)) ;
#62640=DIRECTION('',(1.,0.,2.52374105052742E-18)) ;
#62641=DIRECTION('center_axis',(-0.70710678118661,0.707106781186485,0.)) ;
#62642=DIRECTION('ref_axis',(0.707106781186485,0.70710678118661,3.56910882157392E-18)) ;
#62643=DIRECTION('center_axis',(-1.41426179436738E-51,1.,5.60383084497445E-34)) ;
#62644=DIRECTION('ref_axis',(0.707106781186548,-3.96250679110377E-34,0.707106781186548)) ;
#62645=DIRECTION('',(1.41426179436738E-51,-1.,-5.60383084497445E-34)) ;
#62646=DIRECTION('center_axis',(0.,1.,0.)) ;
#62647=DIRECTION('ref_axis',(1.,0.,2.52374105052742E-18)) ;
#62648=DIRECTION('',(0.,0.,-1.)) ;
#62649=DIRECTION('center_axis',(1.,1.41426179436738E-51,0.)) ;
#62650=DIRECTION('ref_axis',(1.41426179436738E-51,-1.,-5.60383084497445E-34)) ;
#62651=DIRECTION('',(0.,0.,-1.)) ;
#62652=DIRECTION('center_axis',(0.,1.,0.)) ;
#62653=DIRECTION('ref_axis',(1.,0.,2.52374105052742E-18)) ;
#62654=DIRECTION('',(0.,0.,-1.)) ;
#62655=DIRECTION('center_axis',(2.52374105052742E-18,5.60383084497445E-34,
-1.)) ;
#62656=DIRECTION('ref_axis',(1.,3.40207761657885E-68,2.52374105052742E-18)) ;
#62657=DIRECTION('center_axis',(2.52374105052742E-18,5.60383084497445E-34,
-1.)) ;
#62658=DIRECTION('ref_axis',(1.,4.48306467597958E-35,2.52374105052742E-18)) ;
#62659=DIRECTION('center_axis',(2.52374105052742E-18,5.60383084497445E-34,
-1.)) ;
#62660=DIRECTION('ref_axis',(-1.,0.,0.)) ;
#62661=DIRECTION('center_axis',(0.,-1.,-5.60383084497445E-34)) ;
#62662=DIRECTION('ref_axis',(1.,0.,0.)) ;
#62663=DIRECTION('center_axis',(-1.,-1.41426179436738E-51,0.)) ;
#62664=DIRECTION('ref_axis',(-1.41426179436738E-51,1.,5.60383084497445E-34)) ;
#62665=DIRECTION('',(0.,0.,-1.)) ;
#62666=DIRECTION('center_axis',(0.,1.,0.)) ;
#62667=DIRECTION('ref_axis',(1.,0.,2.52374105052742E-18)) ;
#62668=DIRECTION('',(0.,0.,-1.)) ;
#62669=DIRECTION('center_axis',(-1.,-1.41426179436738E-51,0.)) ;
#62670=DIRECTION('ref_axis',(-1.41426179436738E-51,1.,5.60383084497445E-34)) ;
#88392=CARTESIAN_POINT('',(0.,0.,0.)) ;
#88393=CARTESIAN_POINT('Origin',(61.35,261.,30.0213203435596)) ;
#88394=CARTESIAN_POINT('',(61.3,261.,29.9213203435596)) ;
#88395=CARTESIAN_POINT('',(60.1,261.,29.9213203435596)) ;
#88396=CARTESIAN_POINT('',(61.35,261.,29.9213203435596)) ;
#88397=CARTESIAN_POINT('',(60.,260.9,30.0213203435596)) ;
#88398=CARTESIAN_POINT('Origin',(60.1,261.,30.0213203435596)) ;
#88399=CARTESIAN_POINT('',(61.2,260.9,30.0213203435596)) ;
#88400=CARTESIAN_POINT('',(61.35,260.9,30.0213203435596)) ;
#88401=CARTESIAN_POINT('Origin',(61.3,261.,30.0213203435596)) ;
#88402=CARTESIAN_POINT('Origin',(60.1,261.05,30.0213203435596)) ;
#88403=CARTESIAN_POINT('',(60.1,261.4,29.9213203435596)) ;
#88404=CARTESIAN_POINT('',(60.1,261.05,29.9213203435596)) ;
#88405=CARTESIAN_POINT('',(60.,261.5,30.0213203435596)) ;
#88406=CARTESIAN_POINT('Origin',(60.1,261.4,30.0213203435596)) ;
#88407=CARTESIAN_POINT('',(60.,261.05,30.0213203435596)) ;
#88408=CARTESIAN_POINT('Origin',(60.75,261.4,30.0213203435596)) ;
#88409=CARTESIAN_POINT('',(61.3,261.4,29.9213203435596)) ;
#88410=CARTESIAN_POINT('',(60.75,261.4,29.9213203435596)) ;
#88411=CARTESIAN_POINT('',(61.2,261.5,30.0213203435596)) ;
#88412=CARTESIAN_POINT('Origin',(61.3,261.4,30.0213203435596)) ;
#88413=CARTESIAN_POINT('',(60.75,261.5,30.0213203435596)) ;
#88414=CARTESIAN_POINT('Origin',(61.3,261.35,30.0213203435596)) ;
#88415=CARTESIAN_POINT('',(61.3,262.6,29.9213203435596)) ;
#88416=CARTESIAN_POINT('',(61.3,261.35,29.9213203435596)) ;
#88417=CARTESIAN_POINT('',(61.2,262.7,30.0213203435596)) ;
#88418=CARTESIAN_POINT('Origin',(61.3,262.6,30.0213203435596)) ;
#88419=CARTESIAN_POINT('',(61.2,261.35,30.0213203435596)) ;
#88420=CARTESIAN_POINT('Origin',(61.35,262.6,30.0213203435596)) ;
#88421=CARTESIAN_POINT('',(61.7,262.6,29.9213203435596)) ;
#88422=CARTESIAN_POINT('',(61.35,262.6,29.9213203435596)) ;
#88423=CARTESIAN_POINT('',(61.8,262.7,30.0213203435596)) ;
#88424=CARTESIAN_POINT('Origin',(61.7,262.6,30.0213203435596)) ;
#88425=CARTESIAN_POINT('',(61.35,262.7,30.0213203435596)) ;
#88426=CARTESIAN_POINT('Origin',(61.7,261.95,30.0213203435596)) ;
#88427=CARTESIAN_POINT('',(61.8,261.5,30.0213203435596)) ;
#88428=CARTESIAN_POINT('',(61.8,261.95,30.0213203435596)) ;
#88429=CARTESIAN_POINT('',(61.7,261.4,29.9213203435596)) ;
#88430=CARTESIAN_POINT('',(61.7,261.95,29.9213203435596)) ;
#88431=CARTESIAN_POINT('Origin',(61.7,261.4,30.0213203435596)) ;
#88432=CARTESIAN_POINT('Origin',(61.65,261.4,30.0213203435596)) ;
#88433=CARTESIAN_POINT('',(63.,261.5,30.0213203435596)) ;
#88434=CARTESIAN_POINT('',(61.65,261.5,30.0213203435596)) ;
#88435=CARTESIAN_POINT('',(62.9,261.4,29.9213203435596)) ;
#88436=CARTESIAN_POINT('',(61.65,261.4,29.9213203435596)) ;
#88437=CARTESIAN_POINT('Origin',(62.9,261.4,30.0213203435596)) ;
#88438=CARTESIAN_POINT('Origin',(62.9,261.35,30.0213203435596)) ;
#88439=CARTESIAN_POINT('',(63.,260.9,30.0213203435596)) ;
#88440=CARTESIAN_POINT('',(63.,261.35,30.0213203435596)) ;
#88441=CARTESIAN_POINT('',(62.9,261.,29.9213203435596)) ;
#88442=CARTESIAN_POINT('',(62.9,261.35,29.9213203435596)) ;
#88443=CARTESIAN_POINT('Origin',(62.9,261.,30.0213203435596)) ;
#88444=CARTESIAN_POINT('Origin',(62.25,261.,30.0213203435596)) ;
#88445=CARTESIAN_POINT('',(61.8,260.9,30.0213203435596)) ;
#88446=CARTESIAN_POINT('',(62.25,260.9,30.0213203435596)) ;
#88447=CARTESIAN_POINT('',(61.7,261.,29.9213203435596)) ;
#88448=CARTESIAN_POINT('',(62.25,261.,29.9213203435596)) ;
#88449=CARTESIAN_POINT('Origin',(61.7,261.,30.0213203435596)) ;
#88450=CARTESIAN_POINT('Origin',(61.7,261.05,30.0213203435596)) ;
#88451=CARTESIAN_POINT('',(61.8,259.7,30.0213203435596)) ;
#88452=CARTESIAN_POINT('',(61.8,261.05,30.0213203435596)) ;
#88453=CARTESIAN_POINT('',(61.7,259.8,29.9213203435596)) ;
#88454=CARTESIAN_POINT('',(61.7,261.05,29.9213203435596)) ;
#88455=CARTESIAN_POINT('Origin',(61.7,259.8,30.0213203435596)) ;
#88456=CARTESIAN_POINT('Origin',(61.65,259.8,30.0213203435596)) ;
#88457=CARTESIAN_POINT('',(61.2,259.7,30.0213203435596)) ;
#88458=CARTESIAN_POINT('',(61.65,259.7,30.0213203435596)) ;
#88459=CARTESIAN_POINT('',(61.3,259.8,29.9213203435596)) ;
#88460=CARTESIAN_POINT('',(61.65,259.8,29.9213203435596)) ;
#88461=CARTESIAN_POINT('Origin',(61.3,259.8,30.0213203435596)) ;
#88462=CARTESIAN_POINT('Origin',(61.3,260.45,30.0213203435596)) ;
#88463=CARTESIAN_POINT('',(61.2,260.45,30.0213203435596)) ;
#88464=CARTESIAN_POINT('',(61.3,260.45,29.9213203435596)) ;
#88465=CARTESIAN_POINT('Origin',(63.,261.5,30.7213203435596)) ;
#88466=CARTESIAN_POINT('',(63.,260.9,30.1213203435596)) ;
#88467=CARTESIAN_POINT('',(63.,260.9,30.7213203435596)) ;
#88468=CARTESIAN_POINT('',(63.,261.5,30.1213203435596)) ;
#88469=CARTESIAN_POINT('',(63.,261.35,30.1213203435596)) ;
#88470=CARTESIAN_POINT('',(63.,261.5,30.7213203435596)) ;
#88471=CARTESIAN_POINT('Origin',(63.,260.9,30.7213203435596)) ;
#88472=CARTESIAN_POINT('',(61.8,260.9,30.1213203435596)) ;
#88473=CARTESIAN_POINT('',(61.8,260.9,30.7213203435596)) ;
#88474=CARTESIAN_POINT('',(62.25,260.9,30.1213203435596)) ;
#88475=CARTESIAN_POINT('Origin',(61.8,260.9,30.7213203435596)) ;
#88476=CARTESIAN_POINT('',(61.8,259.7,30.1213203435596)) ;
#88477=CARTESIAN_POINT('',(61.8,259.7,30.7213203435596)) ;
#88478=CARTESIAN_POINT('',(61.8,261.05,30.1213203435596)) ;
#88479=CARTESIAN_POINT('Origin',(61.8,259.7,30.7213203435596)) ;
#88480=CARTESIAN_POINT('',(61.2,259.7,30.1213203435596)) ;
#88481=CARTESIAN_POINT('',(61.2,259.7,30.7213203435596)) ;
#88482=CARTESIAN_POINT('',(61.65,259.7,30.1213203435596)) ;
#88483=CARTESIAN_POINT('Origin',(61.2,259.7,30.7213203435596)) ;
#88484=CARTESIAN_POINT('',(61.2,260.9,30.1213203435596)) ;
#88485=CARTESIAN_POINT('',(61.2,260.9,30.7213203435596)) ;
#88486=CARTESIAN_POINT('',(61.2,260.45,30.1213203435596)) ;
#88487=CARTESIAN_POINT('Origin',(61.2,260.9,30.7213203435596)) ;
#88488=CARTESIAN_POINT('',(60.,260.9,30.1213203435596)) ;
#88489=CARTESIAN_POINT('',(60.,260.9,30.7213203435596)) ;
#88490=CARTESIAN_POINT('',(61.35,260.9,30.1213203435596)) ;
#88491=CARTESIAN_POINT('Origin',(61.5,261.2,29.9213203435596)) ;
#88492=CARTESIAN_POINT('Origin',(61.5,261.2,28.8213203435596)) ;
#88493=CARTESIAN_POINT('',(63.9,261.2,28.7213203435596)) ;
#88494=CARTESIAN_POINT('Origin',(61.5,261.2,28.7213203435596)) ;
#88495=CARTESIAN_POINT('',(64.,261.2,28.8213203435596)) ;
#88496=CARTESIAN_POINT('Origin',(63.9,261.2,28.8213203435596)) ;
#88497=CARTESIAN_POINT('',(59.,261.2,28.8213203435596)) ;
#88498=CARTESIAN_POINT('Origin',(61.5,261.2,28.8213203435596)) ;
#88499=CARTESIAN_POINT('Origin',(61.5,261.2,28.8213203435596)) ;
#88500=CARTESIAN_POINT('Origin',(61.5,261.2,30.2213203435596)) ;
#88501=CARTESIAN_POINT('',(59.,261.2,30.0213203435596)) ;
#88502=CARTESIAN_POINT('',(59.,261.2,30.2213203435596)) ;
#88503=CARTESIAN_POINT('',(64.,261.2,30.0213203435596)) ;
#88504=CARTESIAN_POINT('Origin',(61.5,261.2,30.0213203435596)) ;
#88505=CARTESIAN_POINT('Origin',(61.5,261.2,30.0213203435596)) ;
#88506=CARTESIAN_POINT('Origin',(61.5,261.2,28.7213203435596)) ;
#88507=CARTESIAN_POINT('Origin',(61.65,259.6,30.1213203435596)) ;
#88508=CARTESIAN_POINT('',(61.1,259.6,30.2213203435596)) ;
#88509=CARTESIAN_POINT('',(61.9,259.6,30.2213203435596)) ;
#88510=CARTESIAN_POINT('',(61.65,259.6,30.2213203435596)) ;
#88511=CARTESIAN_POINT('Origin',(61.9,259.6,30.1213203435596)) ;
#88512=CARTESIAN_POINT('Origin',(61.1,259.6,30.1213203435596)) ;
#88513=CARTESIAN_POINT('Origin',(61.9,261.05,30.1213203435596)) ;
#88514=CARTESIAN_POINT('',(61.9,260.8,30.2213203435596)) ;
#88515=CARTESIAN_POINT('',(61.9,261.05,30.2213203435596)) ;
#88516=CARTESIAN_POINT('Origin',(61.9,260.8,30.1213203435596)) ;
#88517=CARTESIAN_POINT('Origin',(62.25,260.8,30.1213203435596)) ;
#88518=CARTESIAN_POINT('',(63.1,260.8,30.2213203435596)) ;
#88519=CARTESIAN_POINT('',(62.25,260.8,30.2213203435596)) ;
#88520=CARTESIAN_POINT('Origin',(63.1,260.8,30.1213203435596)) ;
#88521=CARTESIAN_POINT('Origin',(63.1,261.35,30.1213203435596)) ;
#88522=CARTESIAN_POINT('',(63.1,261.6,30.2213203435596)) ;
#88523=CARTESIAN_POINT('',(63.1,261.35,30.2213203435596)) ;
#88524=CARTESIAN_POINT('Origin',(63.1,261.6,30.1213203435596)) ;
#88525=CARTESIAN_POINT('Origin',(61.65,261.6,30.1213203435596)) ;
#88526=CARTESIAN_POINT('',(61.9,261.6,30.2213203435596)) ;
#88527=CARTESIAN_POINT('',(61.65,261.6,30.2213203435596)) ;
#88528=CARTESIAN_POINT('',(61.8,261.5,30.1213203435596)) ;
#88529=CARTESIAN_POINT('Origin',(61.9,261.6,30.1213203435596)) ;
#88530=CARTESIAN_POINT('',(61.65,261.5,30.1213203435596)) ;
#88531=CARTESIAN_POINT('Origin',(61.35,262.8,30.1213203435596)) ;
#88532=CARTESIAN_POINT('',(61.9,262.8,30.2213203435596)) ;
#88533=CARTESIAN_POINT('',(61.1,262.8,30.2213203435596)) ;
#88534=CARTESIAN_POINT('',(61.35,262.8,30.2213203435596)) ;
#88535=CARTESIAN_POINT('',(61.2,262.7,30.1213203435596)) ;
#88536=CARTESIAN_POINT('Origin',(61.1,262.8,30.1213203435596)) ;
#88537=CARTESIAN_POINT('',(61.8,262.7,30.1213203435596)) ;
#88538=CARTESIAN_POINT('',(61.35,262.7,30.1213203435596)) ;
#88539=CARTESIAN_POINT('Origin',(61.9,262.8,30.1213203435596)) ;
#88540=CARTESIAN_POINT('Origin',(61.1,261.35,30.1213203435596)) ;
#88541=CARTESIAN_POINT('',(61.2,261.5,30.1213203435596)) ;
#88542=CARTESIAN_POINT('',(61.2,261.35,30.1213203435596)) ;
#88543=CARTESIAN_POINT('',(61.1,261.6,30.2213203435596)) ;
#88544=CARTESIAN_POINT('',(61.1,261.35,30.2213203435596)) ;
#88545=CARTESIAN_POINT('Origin',(61.1,261.6,30.1213203435596)) ;
#88546=CARTESIAN_POINT('Origin',(61.9,261.95,30.1213203435596)) ;
#88547=CARTESIAN_POINT('',(61.9,261.95,30.2213203435596)) ;
#88548=CARTESIAN_POINT('',(61.8,261.95,30.1213203435596)) ;
#88549=CARTESIAN_POINT('Origin',(60.75,261.6,30.1213203435596)) ;
#88550=CARTESIAN_POINT('',(60.,261.5,30.1213203435596)) ;
#88551=CARTESIAN_POINT('',(60.75,261.5,30.1213203435596)) ;
#88552=CARTESIAN_POINT('',(59.9,261.6,30.2213203435596)) ;
#88553=CARTESIAN_POINT('',(60.75,261.6,30.2213203435596)) ;
#88554=CARTESIAN_POINT('Origin',(59.9,261.6,30.1213203435596)) ;
#88555=CARTESIAN_POINT('Origin',(59.9,261.05,30.1213203435596)) ;
#88556=CARTESIAN_POINT('',(60.,261.05,30.1213203435596)) ;
#88557=CARTESIAN_POINT('',(59.9,260.8,30.2213203435596)) ;
#88558=CARTESIAN_POINT('',(59.9,261.05,30.2213203435596)) ;
#88559=CARTESIAN_POINT('Origin',(59.9,260.8,30.1213203435596)) ;
#88560=CARTESIAN_POINT('Origin',(61.35,260.8,30.1213203435596)) ;
#88561=CARTESIAN_POINT('',(61.1,260.8,30.2213203435596)) ;
#88562=CARTESIAN_POINT('',(61.35,260.8,30.2213203435596)) ;
#88563=CARTESIAN_POINT('Origin',(61.1,260.8,30.1213203435596)) ;
#88564=CARTESIAN_POINT('Origin',(61.1,260.45,30.1213203435596)) ;
#88565=CARTESIAN_POINT('',(61.1,260.45,30.2213203435596)) ;
#88566=CARTESIAN_POINT('Origin',(61.8,261.5,30.7213203435596)) ;
#88567=CARTESIAN_POINT('',(61.8,261.5,30.7213203435596)) ;
#88568=CARTESIAN_POINT('Origin',(61.8,262.7,30.7213203435596)) ;
#88569=CARTESIAN_POINT('',(61.8,262.7,30.7213203435596)) ;
#88570=CARTESIAN_POINT('Origin',(61.2,262.7,30.7213203435596)) ;
#88571=CARTESIAN_POINT('',(61.2,262.7,30.7213203435596)) ;
#88572=CARTESIAN_POINT('Origin',(61.5,261.2,30.2213203435596)) ;
#88573=CARTESIAN_POINT('',(63.8,261.2,30.2213203435596)) ;
#88574=CARTESIAN_POINT('Origin',(61.5,261.2,30.2213203435596)) ;
#88575=CARTESIAN_POINT('Origin',(61.5,261.2,30.0213203435596)) ;
#88576=CARTESIAN_POINT('Origin',(63.8,261.2,30.0213203435596)) ;
#88577=CARTESIAN_POINT('Origin',(60.,260.9,30.7213203435596)) ;
#88578=CARTESIAN_POINT('',(60.,261.5,30.7213203435596)) ;
#88579=CARTESIAN_POINT('Origin',(60.,261.5,30.7213203435596)) ;
#88580=CARTESIAN_POINT('',(61.2,261.5,30.7213203435596)) ;
#88581=CARTESIAN_POINT('Origin',(61.2,261.5,30.7213203435596)) ;
#117138=UNCERTAINTY_MEASURE_WITH_UNIT(LENGTH_MEASURE(0.01),#117171,
'DISTANCE_ACCURACY_VALUE',
'Maximum model space distance between geometric entities at asserted c
onnectivities') ;
#117147=UNCERTAINTY_MEASURE_WITH_UNIT(LENGTH_MEASURE(0.01),#117171,
'DISTANCE_ACCURACY_VALUE',
'Maximum model space distance between geometric entities at asserted c
onnectivities') ;
#117161=(
GEOMETRIC_REPRESENTATION_CONTEXT(3)
GLOBAL_UNCERTAINTY_ASSIGNED_CONTEXT((#117138))
GLOBAL_UNIT_ASSIGNED_CONTEXT((#117171,#117173,#117174))
REPRESENTATION_CONTEXT('','3D')
) ;
#117170=(
GEOMETRIC_REPRESENTATION_CONTEXT(3)
GLOBAL_UNCERTAINTY_ASSIGNED_CONTEXT((#117147))
GLOBAL_UNIT_ASSIGNED_CONTEXT((#117171,#117173,#117174))
REPRESENTATION_CONTEXT('','3D')
) ;
#117171=(
LENGTH_UNIT()
NAMED_UNIT(*)
SI_UNIT(.MILLI.,.METRE.)
) ;
#117173=(
NAMED_UNIT(*)
PLANE_ANGLE_UNIT()
SI_UNIT($,.RADIAN.)
) ;
#117174=(
NAMED_UNIT(*)
SI_UNIT($,.STERADIAN.)
SOLID_ANGLE_UNIT()
) ;
#117188=SHAPE_DEFINITION_REPRESENTATION(#117210,#117253) ;
#117210=PRODUCT_DEFINITION_SHAPE('',$,#117276) ;
#117253=SHAPE_REPRESENTATION('',(#52294),#117161) ;
#117262=PRODUCT_DEFINITION_CONTEXT('part definition',#117330,'design') ;
#117276=PRODUCT_DEFINITION('Spacer_2','Spacer_2',#117298,#117262) ;
#117298=PRODUCT_DEFINITION_FORMATION('',$,#117345) ;
#117330=APPLICATION_CONTEXT(
'Core Data for Automotive Mechanical Design Process') ;
#117331=PRODUCT_CONTEXT('part definition',#117330,'mechanical') ;
#117345=PRODUCT('Spacer_2','Spacer_2',$,(#117331)) ;
#117355=PRESENTATION_STYLE_ASSIGNMENT((#117357)) ;
#117357=SURFACE_STYLE_USAGE(.BOTH.,#117359) ;
#117359=SURFACE_SIDE_STYLE('',(#117361)) ;
#117361=SURFACE_STYLE_FILL_AREA(#117363) ;
#117363=FILL_AREA_STYLE('Opaque(160,160,160)',(#117365)) ;
#117365=FILL_AREA_STYLE_COLOUR('Opaque(160,160,160)',#117367) ;
#117367=COLOUR_RGB('Opaque(160,160,160)', 0.09019608, 0.27058824, 0.51372549) ;
ENDSEC;
END-ISO-10303-21;
